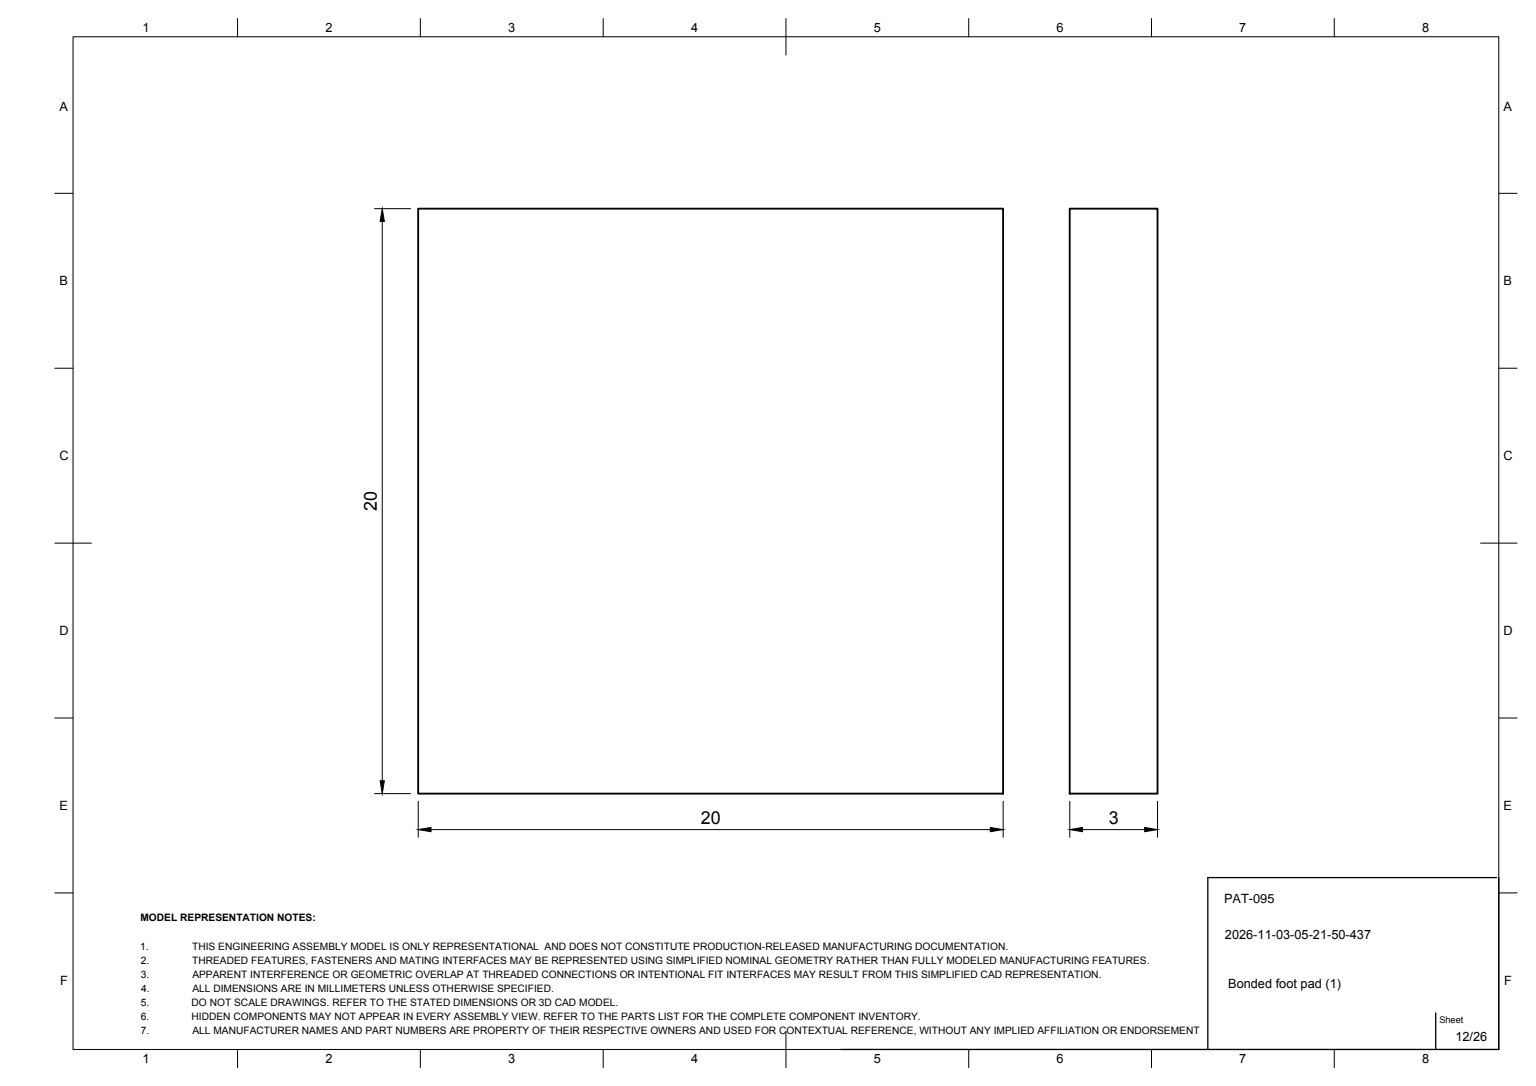
ISO-10303-21;
HEADER;
/* Generated by software containing ST-Developer
 * from STEP Tools, Inc. (www.steptools.com) 
 */

FILE_DESCRIPTION(
/* description */ ('Single-Axis Profile-Rail Linear Slide'),
/* implementation_level */ '2;1');

FILE_NAME(
/* name */ 'Bonded foot pad (1).step',
/* time_stamp */ '2026-10-27T10:47:43-07:00',
/* author */ (''),
/* organization */ (''),
/* preprocessor_version */ 'ST-DEVELOPER v20.2',
/* originating_system */ 'Autodesk Translation Framework v15.17.0.0',
/* authorisation */ '');

FILE_SCHEMA (('AUTOMOTIVE_DESIGN { 1 0 10303 214 3 1 1 }'));
ENDSEC;

DATA;
#10=MECHANICAL_DESIGN_GEOMETRIC_PRESENTATION_REPRESENTATION('',(#336),#14478);
#282=SHAPE_REPRESENTATION_RELATIONSHIP('SRR','None',#14612,#309);
#309=ADVANCED_BREP_SHAPE_REPRESENTATION('',(#363),#14456);
#336=STYLED_ITEM('',(#14824),#363);
#363=MANIFOLD_SOLID_BREP('Body1',#8596);
#630=PLANE('',#9163);
#631=PLANE('',#9164);
#632=PLANE('',#9165);
#633=PLANE('',#9166);
#634=PLANE('',#9167);
#635=PLANE('',#9168);
#1026=FACE_OUTER_BOUND('',#1525,.T.);
#1027=FACE_OUTER_BOUND('',#1526,.T.);
#1028=FACE_OUTER_BOUND('',#1527,.T.);
#1029=FACE_OUTER_BOUND('',#1528,.T.);
#1030=FACE_OUTER_BOUND('',#1529,.T.);
#1031=FACE_OUTER_BOUND('',#1530,.T.);
#1525=EDGE_LOOP('',(#6821,#6822,#6823,#6824));
#1526=EDGE_LOOP('',(#6825,#6826,#6827,#6828));
#1527=EDGE_LOOP('',(#6829,#6830,#6831,#6832));
#1528=EDGE_LOOP('',(#6833,#6834,#6835,#6836));
#1529=EDGE_LOOP('',(#6837,#6838,#6839,#6840));
#1530=EDGE_LOOP('',(#6841,#6842,#6843,#6844));
#2296=LINE('',#13035,#3267);
#2297=LINE('',#13037,#3268);
#2298=LINE('',#13039,#3269);
#2299=LINE('',#13040,#3270);
#2300=LINE('',#13043,#3271);
#2301=LINE('',#13045,#3272);
#2302=LINE('',#13046,#3273);
#2303=LINE('',#13049,#3274);
#2304=LINE('',#13051,#3275);
#2305=LINE('',#13052,#3276);
#2306=LINE('',#13054,#3277);
#2307=LINE('',#13055,#3278);
#3267=VECTOR('',#10567,1.);
#3268=VECTOR('',#10568,1.);
#3269=VECTOR('',#10569,1.);
#3270=VECTOR('',#10570,1.);
#3271=VECTOR('',#10573,1.);
#3272=VECTOR('',#10574,1.);
#3273=VECTOR('',#10575,1.);
#3274=VECTOR('',#10578,1.);
#3275=VECTOR('',#10579,1.);
#3276=VECTOR('',#10580,1.);
#3277=VECTOR('',#10583,1.);
#3278=VECTOR('',#10584,1.);
#4274=VERTEX_POINT('',#13033);
#4275=VERTEX_POINT('',#13034);
#4276=VERTEX_POINT('',#13036);
#4277=VERTEX_POINT('',#13038);
#4278=VERTEX_POINT('',#13042);
#4279=VERTEX_POINT('',#13044);
#4280=VERTEX_POINT('',#13048);
#4281=VERTEX_POINT('',#13050);
#5188=EDGE_CURVE('',#4274,#4275,#2296,.T.);
#5189=EDGE_CURVE('',#4275,#4276,#2297,.T.);
#5190=EDGE_CURVE('',#4277,#4276,#2298,.T.);
#5191=EDGE_CURVE('',#4274,#4277,#2299,.T.);
#5192=EDGE_CURVE('',#4278,#4274,#2300,.T.);
#5193=EDGE_CURVE('',#4279,#4277,#2301,.T.);
#5194=EDGE_CURVE('',#4278,#4279,#2302,.T.);
#5195=EDGE_CURVE('',#4280,#4278,#2303,.T.);
#5196=EDGE_CURVE('',#4281,#4279,#2304,.T.);
#5197=EDGE_CURVE('',#4280,#4281,#2305,.T.);
#5198=EDGE_CURVE('',#4275,#4280,#2306,.T.);
#5199=EDGE_CURVE('',#4276,#4281,#2307,.T.);
#6821=ORIENTED_EDGE('',*,*,#5188,.T.);
#6822=ORIENTED_EDGE('',*,*,#5189,.T.);
#6823=ORIENTED_EDGE('',*,*,#5190,.F.);
#6824=ORIENTED_EDGE('',*,*,#5191,.F.);
#6825=ORIENTED_EDGE('',*,*,#5192,.T.);
#6826=ORIENTED_EDGE('',*,*,#5191,.T.);
#6827=ORIENTED_EDGE('',*,*,#5193,.F.);
#6828=ORIENTED_EDGE('',*,*,#5194,.F.);
#6829=ORIENTED_EDGE('',*,*,#5195,.T.);
#6830=ORIENTED_EDGE('',*,*,#5194,.T.);
#6831=ORIENTED_EDGE('',*,*,#5196,.F.);
#6832=ORIENTED_EDGE('',*,*,#5197,.F.);
#6833=ORIENTED_EDGE('',*,*,#5198,.T.);
#6834=ORIENTED_EDGE('',*,*,#5197,.T.);
#6835=ORIENTED_EDGE('',*,*,#5199,.F.);
#6836=ORIENTED_EDGE('',*,*,#5189,.F.);
#6837=ORIENTED_EDGE('',*,*,#5199,.T.);
#6838=ORIENTED_EDGE('',*,*,#5196,.T.);
#6839=ORIENTED_EDGE('',*,*,#5193,.T.);
#6840=ORIENTED_EDGE('',*,*,#5190,.T.);
#6841=ORIENTED_EDGE('',*,*,#5198,.F.);
#6842=ORIENTED_EDGE('',*,*,#5188,.F.);
#6843=ORIENTED_EDGE('',*,*,#5192,.F.);
#6844=ORIENTED_EDGE('',*,*,#5195,.F.);
#8320=ADVANCED_FACE('',(#1026),#630,.T.);
#8321=ADVANCED_FACE('',(#1027),#631,.T.);
#8322=ADVANCED_FACE('',(#1028),#632,.T.);
#8323=ADVANCED_FACE('',(#1029),#633,.T.);
#8324=ADVANCED_FACE('',(#1030),#634,.T.);
#8325=ADVANCED_FACE('',(#1031),#635,.F.);
#8596=CLOSED_SHELL('',(#8320,#8321,#8322,#8323,#8324,#8325));
#9162=AXIS2_PLACEMENT_3D('',#13031,#10563,#10564);
#9163=AXIS2_PLACEMENT_3D('',#13032,#10565,#10566);
#9164=AXIS2_PLACEMENT_3D('',#13041,#10571,#10572);
#9165=AXIS2_PLACEMENT_3D('',#13047,#10576,#10577);
#9166=AXIS2_PLACEMENT_3D('',#13053,#10581,#10582);
#9167=AXIS2_PLACEMENT_3D('',#13056,#10585,#10586);
#9168=AXIS2_PLACEMENT_3D('',#13057,#10587,#10588);
#10563=DIRECTION('axis',(0.,0.,1.));
#10564=DIRECTION('refdir',(1.,0.,0.));
#10565=DIRECTION('center_axis',(0.,1.,0.));
#10566=DIRECTION('ref_axis',(-1.,0.,0.));
#10567=DIRECTION('',(-1.,0.,0.));
#10568=DIRECTION('',(0.,0.,1.));
#10569=DIRECTION('',(-1.,0.,0.));
#10570=DIRECTION('',(0.,0.,1.));
#10571=DIRECTION('center_axis',(1.,0.,0.));
#10572=DIRECTION('ref_axis',(0.,1.,0.));
#10573=DIRECTION('',(0.,1.,0.));
#10574=DIRECTION('',(0.,1.,0.));
#10575=DIRECTION('',(0.,0.,1.));
#10576=DIRECTION('center_axis',(0.,-1.,0.));
#10577=DIRECTION('ref_axis',(1.,0.,0.));
#10578=DIRECTION('',(1.,0.,0.));
#10579=DIRECTION('',(1.,0.,0.));
#10580=DIRECTION('',(0.,0.,1.));
#10581=DIRECTION('center_axis',(-1.,0.,0.));
#10582=DIRECTION('ref_axis',(0.,-1.,0.));
#10583=DIRECTION('',(0.,-1.,0.));
#10584=DIRECTION('',(0.,-1.,0.));
#10585=DIRECTION('center_axis',(0.,0.,1.));
#10586=DIRECTION('ref_axis',(1.,0.,0.));
#10587=DIRECTION('center_axis',(0.,0.,1.));
#10588=DIRECTION('ref_axis',(1.,0.,0.));
#13031=CARTESIAN_POINT('',(0.,0.,0.));
#13032=CARTESIAN_POINT('Origin',(4.,4.5,-0.3));
#13033=CARTESIAN_POINT('',(4.,4.5,-0.3));
#13034=CARTESIAN_POINT('',(2.,4.5,-0.3));
#13035=CARTESIAN_POINT('',(4.,4.5,-0.3));
#13036=CARTESIAN_POINT('',(2.,4.5,0.));
#13037=CARTESIAN_POINT('',(2.,4.5,-0.3));
#13038=CARTESIAN_POINT('',(4.,4.5,0.));
#13039=CARTESIAN_POINT('',(4.,4.5,0.));
#13040=CARTESIAN_POINT('',(4.,4.5,-0.3));
#13041=CARTESIAN_POINT('Origin',(4.,2.5,-0.3));
#13042=CARTESIAN_POINT('',(4.,2.5,-0.3));
#13043=CARTESIAN_POINT('',(4.,2.5,-0.3));
#13044=CARTESIAN_POINT('',(4.,2.5,0.));
#13045=CARTESIAN_POINT('',(4.,2.5,0.));
#13046=CARTESIAN_POINT('',(4.,2.5,-0.3));
#13047=CARTESIAN_POINT('Origin',(2.,2.5,-0.3));
#13048=CARTESIAN_POINT('',(2.,2.5,-0.3));
#13049=CARTESIAN_POINT('',(2.,2.5,-0.3));
#13050=CARTESIAN_POINT('',(2.,2.5,0.));
#13051=CARTESIAN_POINT('',(2.,2.5,0.));
#13052=CARTESIAN_POINT('',(2.,2.5,-0.3));
#13053=CARTESIAN_POINT('Origin',(2.,4.5,-0.3));
#13054=CARTESIAN_POINT('',(2.,4.5,-0.3));
#13055=CARTESIAN_POINT('',(2.,4.5,0.));
#13056=CARTESIAN_POINT('Origin',(3.,3.5,0.));
#13057=CARTESIAN_POINT('Origin',(3.,3.5,-0.3));
#14424=UNCERTAINTY_MEASURE_WITH_UNIT(LENGTH_MEASURE(0.001),#14479,
'DISTANCE_ACCURACY_VALUE',
'Maximum model space distance between geometric entities at asserted c
onnectivities');
#14446=UNCERTAINTY_MEASURE_WITH_UNIT(LENGTH_MEASURE(0.001),#14479,
'DISTANCE_ACCURACY_VALUE',
'Maximum model space distance between geometric entities at asserted c
onnectivities');
#14456=(
GEOMETRIC_REPRESENTATION_CONTEXT(3)
GLOBAL_UNCERTAINTY_ASSIGNED_CONTEXT((#14424))
GLOBAL_UNIT_ASSIGNED_CONTEXT((#14479,#14481,#14482))
REPRESENTATION_CONTEXT('','3D')
);
#14478=(
GEOMETRIC_REPRESENTATION_CONTEXT(3)
GLOBAL_UNCERTAINTY_ASSIGNED_CONTEXT((#14446))
GLOBAL_UNIT_ASSIGNED_CONTEXT((#14479,#14481,#14482))
REPRESENTATION_CONTEXT('','3D')
);
#14479=(
LENGTH_UNIT()
NAMED_UNIT(*)
SI_UNIT(.CENTI.,.METRE.)
);
#14481=(
NAMED_UNIT(*)
PLANE_ANGLE_UNIT()
SI_UNIT($,.RADIAN.)
);
#14482=(
NAMED_UNIT(*)
SI_UNIT($,.STERADIAN.)
SOLID_ANGLE_UNIT()
);
#14492=SHAPE_DEFINITION_REPRESENTATION(#14523,#14612);
#14523=PRODUCT_DEFINITION_SHAPE('',$,#14644);
#14612=SHAPE_REPRESENTATION('',(#9162),#14456);
#14634=PRODUCT_DEFINITION_CONTEXT('part definition',#14729,'design');
#14644=PRODUCT_DEFINITION('Bonded foot pad (1)','Bonded foot pad (1)',#14675,
#14634);
#14675=PRODUCT_DEFINITION_FORMATION('',$,#14740);
#14729=APPLICATION_CONTEXT(
'Core Data for Automotive Mechanical Design Process');
#14730=PRODUCT_CONTEXT('part definition',#14729,'mechanical');
#14740=PRODUCT('Bonded foot pad (1)','Bonded foot pad (1)',
'Bonded foot pad (1)',(#14730));
#14818=COLOUR_RGB('Sky Blue',0.24,0.69,0.87);
#14819=FILL_AREA_STYLE_COLOUR('',#14818);
#14820=FILL_AREA_STYLE('',(#14819));
#14821=SURFACE_STYLE_FILL_AREA(#14820);
#14822=SURFACE_SIDE_STYLE('',(#14821));
#14823=SURFACE_STYLE_USAGE(.BOTH.,#14822);
#14824=PRESENTATION_STYLE_ASSIGNMENT((#14823));
ENDSEC;
END-ISO-10303-21;
